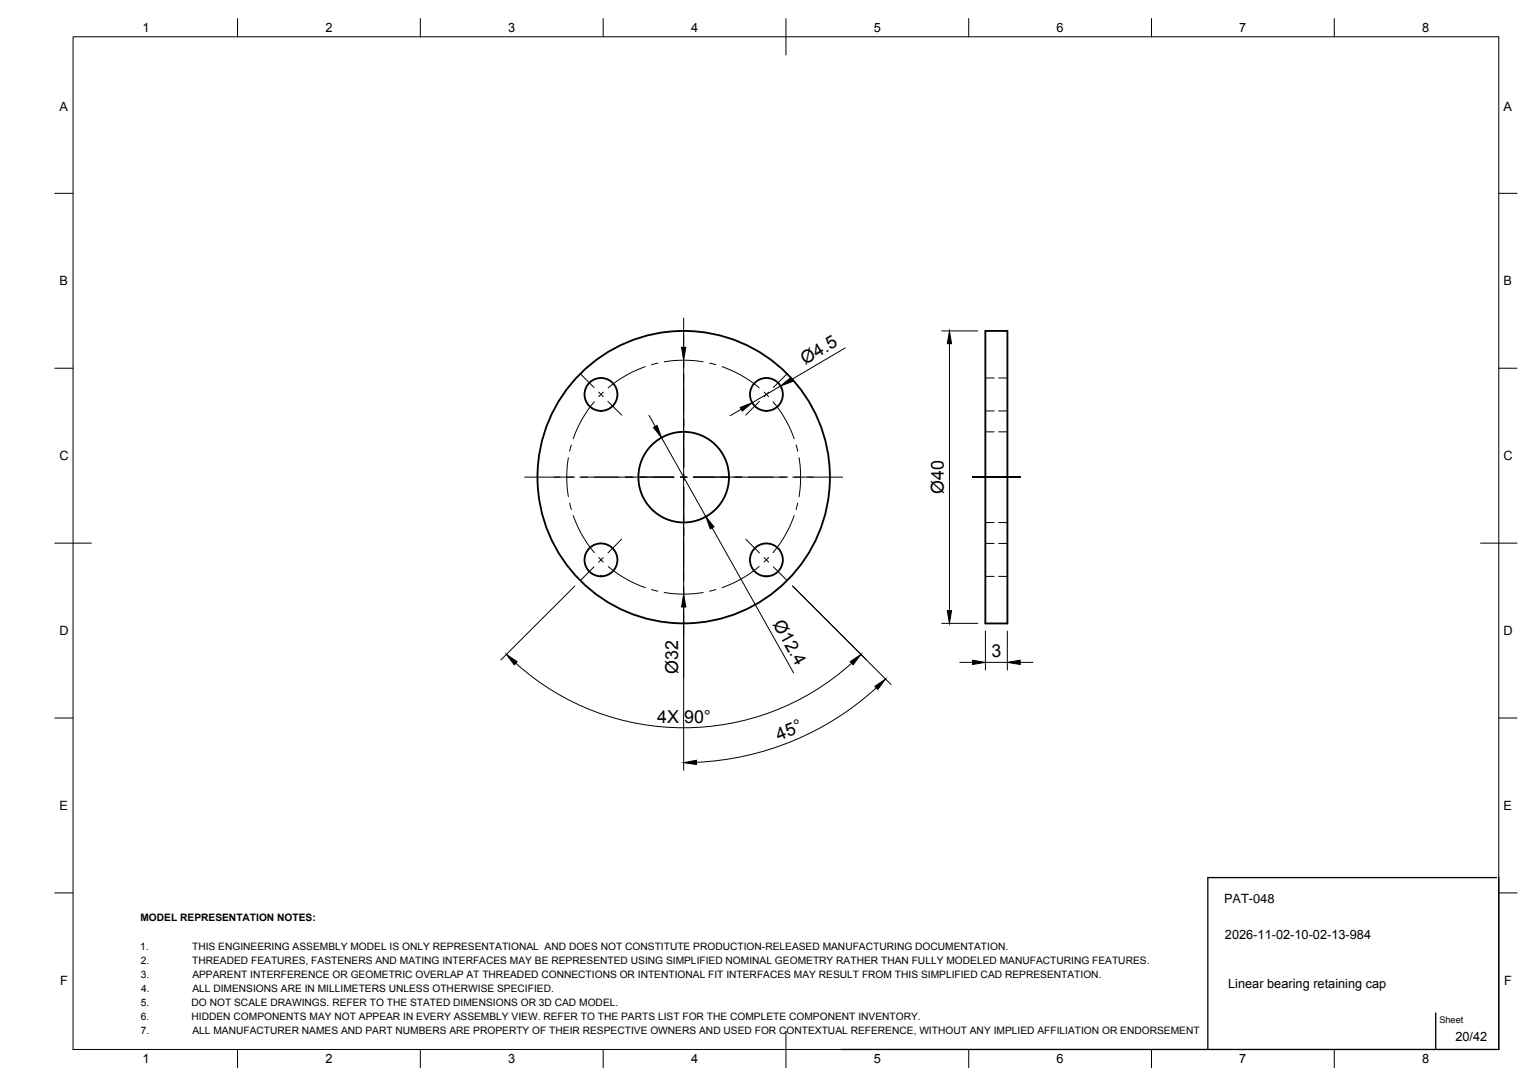
ISO-10303-21;
HEADER;
/* Generated by software containing ST-Developer
 * from STEP Tools, Inc. (www.steptools.com) 
 */

FILE_DESCRIPTION(
/* description */ ('Guided pneumatic stop gate'),
/* implementation_level */ '2;1');

FILE_NAME(
/* name */ 'Linear bearing retaining cap.step',
/* time_stamp */ '2026-10-27T21:43:45-07:00',
/* author */ (''),
/* organization */ (''),
/* preprocessor_version */ 'ST-DEVELOPER v20.2',
/* originating_system */ 'Autodesk Translation Framework v15.17.0.0',
/* authorisation */ '');

FILE_SCHEMA (('AUTOMOTIVE_DESIGN { 1 0 10303 214 3 1 1 }'));
ENDSEC;

DATA;
#10=MECHANICAL_DESIGN_GEOMETRIC_PRESENTATION_REPRESENTATION('',(#555),#14392);
#471=SHAPE_REPRESENTATION_RELATIONSHIP('SRR','None',#14606,#513);
#513=ADVANCED_BREP_SHAPE_REPRESENTATION('',(#596),#14368);
#555=STYLED_ITEM('',(#14891),#596);
#596=MANIFOLD_SOLID_BREP('Body1',#7896);
#737=FACE_BOUND('',#1988,.T.);
#738=FACE_BOUND('',#1989,.T.);
#739=FACE_BOUND('',#1990,.T.);
#740=FACE_BOUND('',#1991,.T.);
#741=FACE_BOUND('',#1992,.T.);
#742=FACE_BOUND('',#1994,.T.);
#743=FACE_BOUND('',#1995,.T.);
#744=FACE_BOUND('',#1996,.T.);
#745=FACE_BOUND('',#1997,.T.);
#746=FACE_BOUND('',#1998,.T.);
#995=PLANE('',#8915);
#996=PLANE('',#8916);
#1384=FACE_OUTER_BOUND('',#1981,.T.);
#1385=FACE_OUTER_BOUND('',#1982,.T.);
#1386=FACE_OUTER_BOUND('',#1983,.T.);
#1387=FACE_OUTER_BOUND('',#1984,.T.);
#1388=FACE_OUTER_BOUND('',#1985,.T.);
#1389=FACE_OUTER_BOUND('',#1986,.T.);
#1390=FACE_OUTER_BOUND('',#1987,.T.);
#1391=FACE_OUTER_BOUND('',#1993,.T.);
#1981=EDGE_LOOP('',(#6402,#6403,#6404,#6405));
#1982=EDGE_LOOP('',(#6406,#6407,#6408,#6409));
#1983=EDGE_LOOP('',(#6410,#6411,#6412,#6413));
#1984=EDGE_LOOP('',(#6414,#6415,#6416,#6417));
#1985=EDGE_LOOP('',(#6418,#6419,#6420,#6421));
#1986=EDGE_LOOP('',(#6422,#6423,#6424,#6425));
#1987=EDGE_LOOP('',(#6426));
#1988=EDGE_LOOP('',(#6427));
#1989=EDGE_LOOP('',(#6428));
#1990=EDGE_LOOP('',(#6429));
#1991=EDGE_LOOP('',(#6430));
#1992=EDGE_LOOP('',(#6431));
#1993=EDGE_LOOP('',(#6432));
#1994=EDGE_LOOP('',(#6433));
#1995=EDGE_LOOP('',(#6434));
#1996=EDGE_LOOP('',(#6435));
#1997=EDGE_LOOP('',(#6436));
#1998=EDGE_LOOP('',(#6437));
#2588=LINE('',#13130,#3133);
#2589=LINE('',#13136,#3134);
#2590=LINE('',#13142,#3135);
#2591=LINE('',#13148,#3136);
#2592=LINE('',#13154,#3137);
#2593=LINE('',#13160,#3138);
#3133=VECTOR('',#10721,0.225);
#3134=VECTOR('',#10728,0.225);
#3135=VECTOR('',#10735,0.225);
#3136=VECTOR('',#10742,0.225);
#3137=VECTOR('',#10749,0.62);
#3138=VECTOR('',#10756,2.);
#3575=CIRCLE('',#8898,0.225);
#3576=CIRCLE('',#8899,0.225);
#3577=CIRCLE('',#8901,0.225);
#3578=CIRCLE('',#8902,0.225);
#3579=CIRCLE('',#8904,0.225);
#3580=CIRCLE('',#8905,0.225);
#3581=CIRCLE('',#8907,0.225);
#3582=CIRCLE('',#8908,0.225);
#3583=CIRCLE('',#8910,0.62);
#3584=CIRCLE('',#8911,0.62);
#3585=CIRCLE('',#8913,2.);
#3586=CIRCLE('',#8914,2.);
#4084=VERTEX_POINT('',#13127);
#4085=VERTEX_POINT('',#13129);
#4086=VERTEX_POINT('',#13133);
#4087=VERTEX_POINT('',#13135);
#4088=VERTEX_POINT('',#13139);
#4089=VERTEX_POINT('',#13141);
#4090=VERTEX_POINT('',#13145);
#4091=VERTEX_POINT('',#13147);
#4092=VERTEX_POINT('',#13151);
#4093=VERTEX_POINT('',#13153);
#4094=VERTEX_POINT('',#13157);
#4095=VERTEX_POINT('',#13159);
#4899=EDGE_CURVE('',#4084,#4084,#3575,.T.);
#4900=EDGE_CURVE('',#4084,#4085,#2588,.T.);
#4901=EDGE_CURVE('',#4085,#4085,#3576,.T.);
#4902=EDGE_CURVE('',#4086,#4086,#3577,.T.);
#4903=EDGE_CURVE('',#4086,#4087,#2589,.T.);
#4904=EDGE_CURVE('',#4087,#4087,#3578,.T.);
#4905=EDGE_CURVE('',#4088,#4088,#3579,.T.);
#4906=EDGE_CURVE('',#4088,#4089,#2590,.T.);
#4907=EDGE_CURVE('',#4089,#4089,#3580,.T.);
#4908=EDGE_CURVE('',#4090,#4090,#3581,.T.);
#4909=EDGE_CURVE('',#4090,#4091,#2591,.T.);
#4910=EDGE_CURVE('',#4091,#4091,#3582,.T.);
#4911=EDGE_CURVE('',#4092,#4092,#3583,.T.);
#4912=EDGE_CURVE('',#4092,#4093,#2592,.T.);
#4913=EDGE_CURVE('',#4093,#4093,#3584,.T.);
#4914=EDGE_CURVE('',#4094,#4094,#3585,.T.);
#4915=EDGE_CURVE('',#4094,#4095,#2593,.T.);
#4916=EDGE_CURVE('',#4095,#4095,#3586,.T.);
#6402=ORIENTED_EDGE('',*,*,#4899,.F.);
#6403=ORIENTED_EDGE('',*,*,#4900,.T.);
#6404=ORIENTED_EDGE('',*,*,#4901,.F.);
#6405=ORIENTED_EDGE('',*,*,#4900,.F.);
#6406=ORIENTED_EDGE('',*,*,#4902,.F.);
#6407=ORIENTED_EDGE('',*,*,#4903,.T.);
#6408=ORIENTED_EDGE('',*,*,#4904,.F.);
#6409=ORIENTED_EDGE('',*,*,#4903,.F.);
#6410=ORIENTED_EDGE('',*,*,#4905,.F.);
#6411=ORIENTED_EDGE('',*,*,#4906,.T.);
#6412=ORIENTED_EDGE('',*,*,#4907,.F.);
#6413=ORIENTED_EDGE('',*,*,#4906,.F.);
#6414=ORIENTED_EDGE('',*,*,#4908,.F.);
#6415=ORIENTED_EDGE('',*,*,#4909,.T.);
#6416=ORIENTED_EDGE('',*,*,#4910,.F.);
#6417=ORIENTED_EDGE('',*,*,#4909,.F.);
#6418=ORIENTED_EDGE('',*,*,#4911,.F.);
#6419=ORIENTED_EDGE('',*,*,#4912,.T.);
#6420=ORIENTED_EDGE('',*,*,#4913,.T.);
#6421=ORIENTED_EDGE('',*,*,#4912,.F.);
#6422=ORIENTED_EDGE('',*,*,#4914,.F.);
#6423=ORIENTED_EDGE('',*,*,#4915,.T.);
#6424=ORIENTED_EDGE('',*,*,#4916,.T.);
#6425=ORIENTED_EDGE('',*,*,#4915,.F.);
#6426=ORIENTED_EDGE('',*,*,#4914,.T.);
#6427=ORIENTED_EDGE('',*,*,#4911,.T.);
#6428=ORIENTED_EDGE('',*,*,#4910,.T.);
#6429=ORIENTED_EDGE('',*,*,#4907,.T.);
#6430=ORIENTED_EDGE('',*,*,#4904,.T.);
#6431=ORIENTED_EDGE('',*,*,#4901,.T.);
#6432=ORIENTED_EDGE('',*,*,#4916,.F.);
#6433=ORIENTED_EDGE('',*,*,#4913,.F.);
#6434=ORIENTED_EDGE('',*,*,#4908,.T.);
#6435=ORIENTED_EDGE('',*,*,#4905,.T.);
#6436=ORIENTED_EDGE('',*,*,#4902,.T.);
#6437=ORIENTED_EDGE('',*,*,#4899,.T.);
#7333=CYLINDRICAL_SURFACE('',#8897,0.225);
#7334=CYLINDRICAL_SURFACE('',#8900,0.225);
#7335=CYLINDRICAL_SURFACE('',#8903,0.225);
#7336=CYLINDRICAL_SURFACE('',#8906,0.225);
#7337=CYLINDRICAL_SURFACE('',#8909,0.62);
#7338=CYLINDRICAL_SURFACE('',#8912,2.);
#7666=ADVANCED_FACE('',(#1384),#7333,.F.);
#7667=ADVANCED_FACE('',(#1385),#7334,.F.);
#7668=ADVANCED_FACE('',(#1386),#7335,.F.);
#7669=ADVANCED_FACE('',(#1387),#7336,.F.);
#7670=ADVANCED_FACE('',(#1388),#7337,.F.);
#7671=ADVANCED_FACE('',(#1389),#7338,.T.);
#7672=ADVANCED_FACE('',(#1390,#737,#738,#739,#740,#741),#995,.T.);
#7673=ADVANCED_FACE('',(#1391,#742,#743,#744,#745,#746),#996,.F.);
#7896=CLOSED_SHELL('',(#7666,#7667,#7668,#7669,#7670,#7671,#7672,#7673));
#8896=AXIS2_PLACEMENT_3D('',#13125,#10715,#10716);
#8897=AXIS2_PLACEMENT_3D('',#13126,#10717,#10718);
#8898=AXIS2_PLACEMENT_3D('',#13128,#10719,#10720);
#8899=AXIS2_PLACEMENT_3D('',#13131,#10722,#10723);
#8900=AXIS2_PLACEMENT_3D('',#13132,#10724,#10725);
#8901=AXIS2_PLACEMENT_3D('',#13134,#10726,#10727);
#8902=AXIS2_PLACEMENT_3D('',#13137,#10729,#10730);
#8903=AXIS2_PLACEMENT_3D('',#13138,#10731,#10732);
#8904=AXIS2_PLACEMENT_3D('',#13140,#10733,#10734);
#8905=AXIS2_PLACEMENT_3D('',#13143,#10736,#10737);
#8906=AXIS2_PLACEMENT_3D('',#13144,#10738,#10739);
#8907=AXIS2_PLACEMENT_3D('',#13146,#10740,#10741);
#8908=AXIS2_PLACEMENT_3D('',#13149,#10743,#10744);
#8909=AXIS2_PLACEMENT_3D('',#13150,#10745,#10746);
#8910=AXIS2_PLACEMENT_3D('',#13152,#10747,#10748);
#8911=AXIS2_PLACEMENT_3D('',#13155,#10750,#10751);
#8912=AXIS2_PLACEMENT_3D('',#13156,#10752,#10753);
#8913=AXIS2_PLACEMENT_3D('',#13158,#10754,#10755);
#8914=AXIS2_PLACEMENT_3D('',#13161,#10757,#10758);
#8915=AXIS2_PLACEMENT_3D('',#13162,#10759,#10760);
#8916=AXIS2_PLACEMENT_3D('',#13163,#10761,#10762);
#10715=DIRECTION('axis',(0.,0.,1.));
#10716=DIRECTION('refdir',(1.,0.,0.));
#10717=DIRECTION('center_axis',(0.,1.,0.));
#10718=DIRECTION('ref_axis',(1.,0.,0.));
#10719=DIRECTION('center_axis',(0.,1.,0.));
#10720=DIRECTION('ref_axis',(1.,0.,0.));
#10721=DIRECTION('',(0.,1.,0.));
#10722=DIRECTION('center_axis',(0.,-1.,0.));
#10723=DIRECTION('ref_axis',(1.,0.,0.));
#10724=DIRECTION('center_axis',(0.,1.,0.));
#10725=DIRECTION('ref_axis',(1.,0.,0.));
#10726=DIRECTION('center_axis',(0.,1.,0.));
#10727=DIRECTION('ref_axis',(1.,0.,0.));
#10728=DIRECTION('',(0.,1.,0.));
#10729=DIRECTION('center_axis',(0.,-1.,0.));
#10730=DIRECTION('ref_axis',(1.,0.,0.));
#10731=DIRECTION('center_axis',(0.,1.,0.));
#10732=DIRECTION('ref_axis',(1.,0.,0.));
#10733=DIRECTION('center_axis',(0.,1.,0.));
#10734=DIRECTION('ref_axis',(1.,0.,0.));
#10735=DIRECTION('',(0.,1.,0.));
#10736=DIRECTION('center_axis',(0.,-1.,0.));
#10737=DIRECTION('ref_axis',(1.,0.,0.));
#10738=DIRECTION('center_axis',(0.,1.,0.));
#10739=DIRECTION('ref_axis',(1.,0.,0.));
#10740=DIRECTION('center_axis',(0.,1.,0.));
#10741=DIRECTION('ref_axis',(1.,0.,0.));
#10742=DIRECTION('',(0.,1.,0.));
#10743=DIRECTION('center_axis',(0.,-1.,0.));
#10744=DIRECTION('ref_axis',(1.,0.,0.));
#10745=DIRECTION('center_axis',(0.,1.,0.));
#10746=DIRECTION('ref_axis',(1.,0.,0.));
#10747=DIRECTION('center_axis',(0.,-1.,0.));
#10748=DIRECTION('ref_axis',(1.,0.,0.));
#10749=DIRECTION('',(0.,-1.,0.));
#10750=DIRECTION('center_axis',(0.,-1.,0.));
#10751=DIRECTION('ref_axis',(1.,0.,0.));
#10752=DIRECTION('center_axis',(0.,1.,0.));
#10753=DIRECTION('ref_axis',(1.,0.,0.));
#10754=DIRECTION('center_axis',(0.,1.,0.));
#10755=DIRECTION('ref_axis',(1.,0.,0.));
#10756=DIRECTION('',(0.,-1.,0.));
#10757=DIRECTION('center_axis',(0.,1.,0.));
#10758=DIRECTION('ref_axis',(1.,0.,0.));
#10759=DIRECTION('center_axis',(0.,1.,0.));
#10760=DIRECTION('ref_axis',(1.,0.,0.));
#10761=DIRECTION('center_axis',(0.,1.,0.));
#10762=DIRECTION('ref_axis',(1.,0.,0.));
#13125=CARTESIAN_POINT('',(0.,0.,0.));
#13126=CARTESIAN_POINT('Origin',(-6.13137084989848,5.6,3.36862915010152));
#13127=CARTESIAN_POINT('',(-6.35637084989848,5.7,3.36862915010152));
#13128=CARTESIAN_POINT('Origin',(-6.13137084989848,5.7,3.36862915010152));
#13129=CARTESIAN_POINT('',(-6.35637084989848,6.,3.36862915010152));
#13130=CARTESIAN_POINT('',(-6.35637084989848,5.6,3.36862915010152));
#13131=CARTESIAN_POINT('Origin',(-6.13137084989848,6.,3.36862915010152));
#13132=CARTESIAN_POINT('Origin',(-6.13137084989848,5.6,5.63137084989848));
#13133=CARTESIAN_POINT('',(-6.35637084989848,5.7,5.63137084989848));
#13134=CARTESIAN_POINT('Origin',(-6.13137084989848,5.7,5.63137084989848));
#13135=CARTESIAN_POINT('',(-6.35637084989848,6.,5.63137084989848));
#13136=CARTESIAN_POINT('',(-6.35637084989848,5.6,5.63137084989848));
#13137=CARTESIAN_POINT('Origin',(-6.13137084989848,6.,5.63137084989848));
#13138=CARTESIAN_POINT('Origin',(-3.86862915010152,5.6,5.63137084989848));
#13139=CARTESIAN_POINT('',(-4.09362915010152,5.7,5.63137084989848));
#13140=CARTESIAN_POINT('Origin',(-3.86862915010152,5.7,5.63137084989848));
#13141=CARTESIAN_POINT('',(-4.09362915010152,6.,5.63137084989848));
#13142=CARTESIAN_POINT('',(-4.09362915010152,5.6,5.63137084989848));
#13143=CARTESIAN_POINT('Origin',(-3.86862915010152,6.,5.63137084989848));
#13144=CARTESIAN_POINT('Origin',(-3.86862915010152,5.6,3.36862915010152));
#13145=CARTESIAN_POINT('',(-4.09362915010152,5.7,3.36862915010152));
#13146=CARTESIAN_POINT('Origin',(-3.86862915010152,5.7,3.36862915010152));
#13147=CARTESIAN_POINT('',(-4.09362915010152,6.,3.36862915010152));
#13148=CARTESIAN_POINT('',(-4.09362915010152,5.6,3.36862915010152));
#13149=CARTESIAN_POINT('Origin',(-3.86862915010152,6.,3.36862915010152));
#13150=CARTESIAN_POINT('Origin',(-5.,5.7,4.5));
#13151=CARTESIAN_POINT('',(-5.62,6.,4.5));
#13152=CARTESIAN_POINT('Origin',(-5.,6.,4.5));
#13153=CARTESIAN_POINT('',(-5.62,5.7,4.5));
#13154=CARTESIAN_POINT('',(-5.62,5.7,4.5));
#13155=CARTESIAN_POINT('Origin',(-5.,5.7,4.5));
#13156=CARTESIAN_POINT('Origin',(-5.,5.7,4.5));
#13157=CARTESIAN_POINT('',(-7.,6.,4.5));
#13158=CARTESIAN_POINT('Origin',(-5.,6.,4.5));
#13159=CARTESIAN_POINT('',(-7.,5.7,4.5));
#13160=CARTESIAN_POINT('',(-7.,5.7,4.5));
#13161=CARTESIAN_POINT('Origin',(-5.,5.7,4.5));
#13162=CARTESIAN_POINT('Origin',(-5.,6.,4.5));
#13163=CARTESIAN_POINT('Origin',(-5.,5.7,4.5));
#14320=UNCERTAINTY_MEASURE_WITH_UNIT(LENGTH_MEASURE(0.001),#14393,
'DISTANCE_ACCURACY_VALUE',
'Maximum model space distance between geometric entities at asserted c
onnectivities');
#14344=UNCERTAINTY_MEASURE_WITH_UNIT(LENGTH_MEASURE(0.001),#14393,
'DISTANCE_ACCURACY_VALUE',
'Maximum model space distance between geometric entities at asserted c
onnectivities');
#14368=(
GEOMETRIC_REPRESENTATION_CONTEXT(3)
GLOBAL_UNCERTAINTY_ASSIGNED_CONTEXT((#14320))
GLOBAL_UNIT_ASSIGNED_CONTEXT((#14393,#14395,#14396))
REPRESENTATION_CONTEXT('','3D')
);
#14392=(
GEOMETRIC_REPRESENTATION_CONTEXT(3)
GLOBAL_UNCERTAINTY_ASSIGNED_CONTEXT((#14344))
GLOBAL_UNIT_ASSIGNED_CONTEXT((#14393,#14395,#14396))
REPRESENTATION_CONTEXT('','3D')
);
#14393=(
LENGTH_UNIT()
NAMED_UNIT(*)
SI_UNIT(.CENTI.,.METRE.)
);
#14395=(
NAMED_UNIT(*)
PLANE_ANGLE_UNIT()
SI_UNIT($,.RADIAN.)
);
#14396=(
NAMED_UNIT(*)
SI_UNIT($,.STERADIAN.)
SOLID_ANGLE_UNIT()
);
#14420=SHAPE_DEFINITION_REPRESENTATION(#14469,#14606);
#14469=PRODUCT_DEFINITION_SHAPE('',$,#14654);
#14606=SHAPE_REPRESENTATION('',(#8896),#14368);
#14630=PRODUCT_DEFINITION_CONTEXT('part definition',#14773,'design');
#14654=PRODUCT_DEFINITION('Linear bearing retaining cap',
'Linear bearing retaining cap',#14701,#14630);
#14701=PRODUCT_DEFINITION_FORMATION('',$,#14798);
#14773=APPLICATION_CONTEXT(
'Core Data for Automotive Mechanical Design Process');
#14774=PRODUCT_CONTEXT('part definition',#14773,'mechanical');
#14798=PRODUCT('Linear bearing retaining cap',
'Linear bearing retaining cap','Linear bearing retaining cap',(#14774));
#14885=COLOUR_RGB('Grey',0.48,0.52,0.57);
#14886=FILL_AREA_STYLE_COLOUR('',#14885);
#14887=FILL_AREA_STYLE('',(#14886));
#14888=SURFACE_STYLE_FILL_AREA(#14887);
#14889=SURFACE_SIDE_STYLE('',(#14888));
#14890=SURFACE_STYLE_USAGE(.BOTH.,#14889);
#14891=PRESENTATION_STYLE_ASSIGNMENT((#14890));
ENDSEC;
END-ISO-10303-21;
